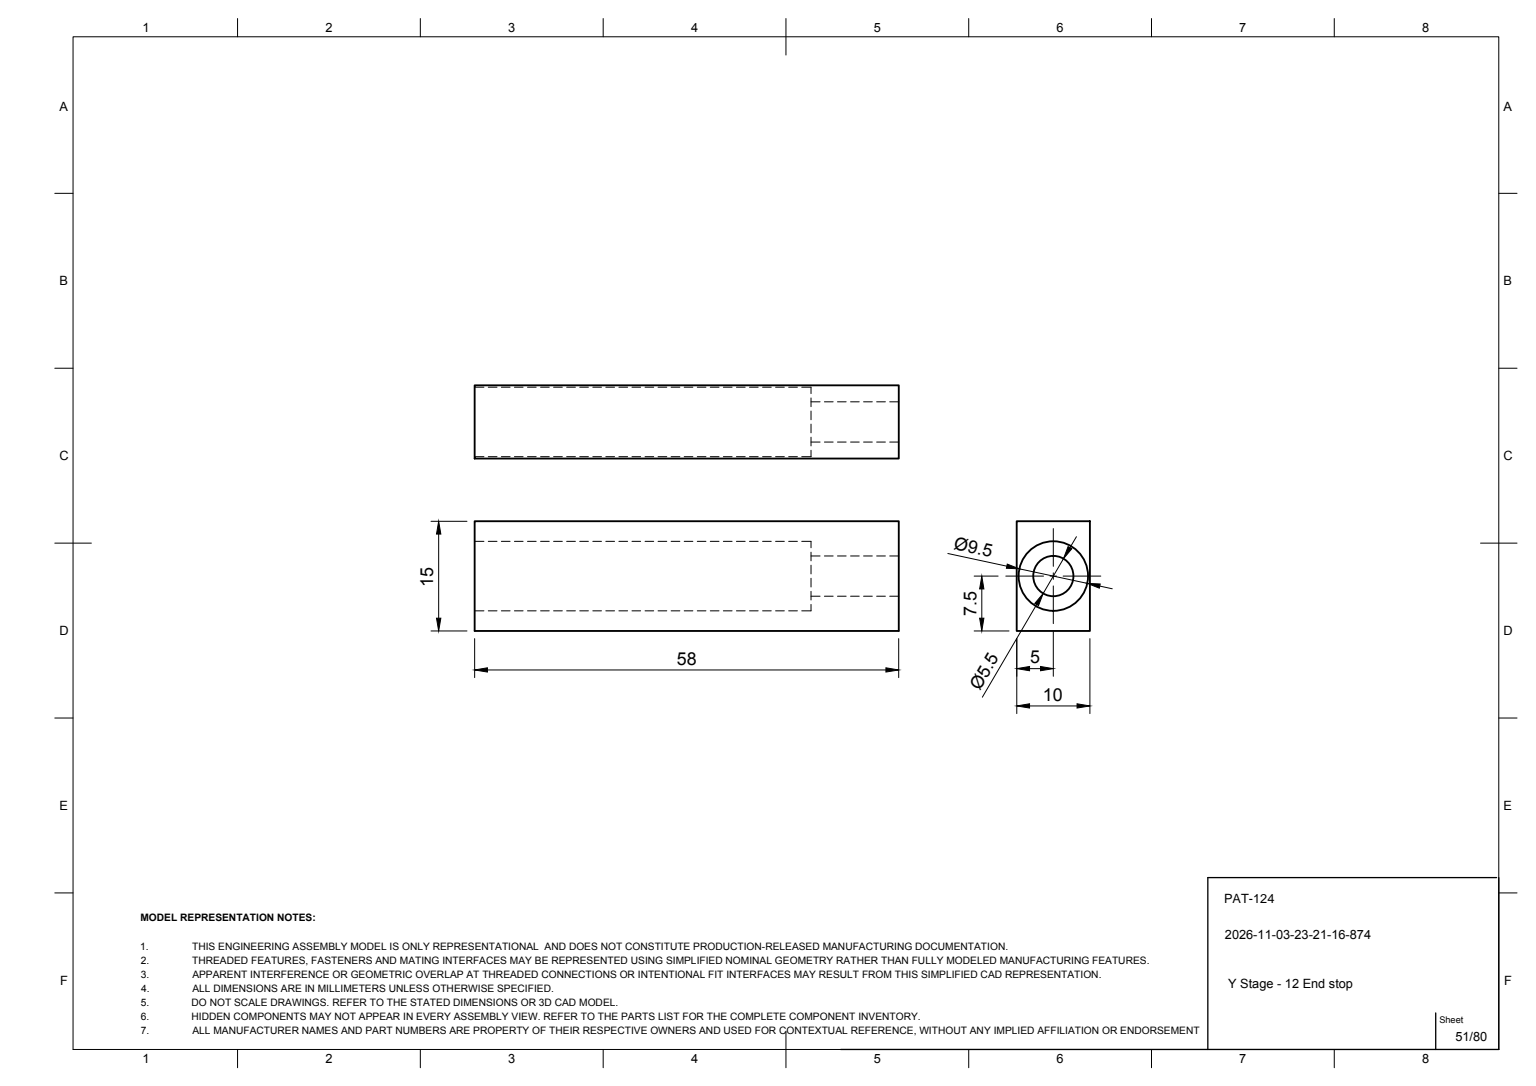
ISO-10303-21;
HEADER;
/* Generated by software containing ST-Developer
 * from STEP Tools, Inc. (www.steptools.com) 
 */

FILE_DESCRIPTION(
/* description */ ('XY cross-slide table'),
/* implementation_level */ '2;1');

FILE_NAME(
/* name */ 'Y Stage - 12 End stop.step',
/* time_stamp */ '2026-10-28T03:22:46-07:00',
/* author */ (''),
/* organization */ (''),
/* preprocessor_version */ 'ST-DEVELOPER v20.2',
/* originating_system */ 'Autodesk Translation Framework v15.17.0.0',
/* authorisation */ '');

FILE_SCHEMA (('AUTOMOTIVE_DESIGN { 1 0 10303 214 3 1 1 }'));
ENDSEC;

DATA;
#10=MECHANICAL_DESIGN_GEOMETRIC_PRESENTATION_REPRESENTATION('',(#1733),#62984);
#1552=SHAPE_REPRESENTATION_RELATIONSHIP('SRR','None',#63407,#1635);
#1635=ADVANCED_BREP_SHAPE_REPRESENTATION('',(#1842),#62944);
#1733=STYLED_ITEM('',(#63905),#1842);
#1842=MANIFOLD_SOLID_BREP('Body1',#23031);
#2183=FACE_BOUND('',#5243,.T.);
#2184=FACE_BOUND('',#5250,.T.);
#2185=FACE_BOUND('',#5252,.T.);
#2630=PLANE('',#25463);
#2631=PLANE('',#25467);
#2632=PLANE('',#25468);
#2633=PLANE('',#25469);
#2634=PLANE('',#25470);
#2635=PLANE('',#25471);
#2636=PLANE('',#25472);
#3631=FACE_OUTER_BOUND('',#5241,.T.);
#3632=FACE_OUTER_BOUND('',#5242,.T.);
#3633=FACE_OUTER_BOUND('',#5244,.T.);
#3634=FACE_OUTER_BOUND('',#5245,.T.);
#3635=FACE_OUTER_BOUND('',#5246,.T.);
#3636=FACE_OUTER_BOUND('',#5247,.T.);
#3637=FACE_OUTER_BOUND('',#5248,.T.);
#3638=FACE_OUTER_BOUND('',#5249,.T.);
#3639=FACE_OUTER_BOUND('',#5251,.T.);
#5241=EDGE_LOOP('',(#18436,#18437,#18438,#18439));
#5242=EDGE_LOOP('',(#18440));
#5243=EDGE_LOOP('',(#18441));
#5244=EDGE_LOOP('',(#18442,#18443,#18444,#18445));
#5245=EDGE_LOOP('',(#18446,#18447,#18448,#18449));
#5246=EDGE_LOOP('',(#18450,#18451,#18452,#18453));
#5247=EDGE_LOOP('',(#18454,#18455,#18456,#18457));
#5248=EDGE_LOOP('',(#18458,#18459,#18460,#18461));
#5249=EDGE_LOOP('',(#18462,#18463,#18464,#18465));
#5250=EDGE_LOOP('',(#18466));
#5251=EDGE_LOOP('',(#18467,#18468,#18469,#18470));
#5252=EDGE_LOOP('',(#18471));
#6765=LINE('',#48330,#8252);
#6766=LINE('',#48338,#8253);
#6767=LINE('',#48342,#8254);
#6768=LINE('',#48344,#8255);
#6769=LINE('',#48346,#8256);
#6770=LINE('',#48347,#8257);
#6771=LINE('',#48350,#8258);
#6772=LINE('',#48352,#8259);
#6773=LINE('',#48353,#8260);
#6774=LINE('',#48356,#8261);
#6775=LINE('',#48358,#8262);
#6776=LINE('',#48359,#8263);
#6777=LINE('',#48361,#8264);
#6778=LINE('',#48362,#8265);
#8252=VECTOR('',#30244,0.475);
#8253=VECTOR('',#30255,0.275);
#8254=VECTOR('',#30258,1.);
#8255=VECTOR('',#30259,1.);
#8256=VECTOR('',#30260,1.);
#8257=VECTOR('',#30261,1.);
#8258=VECTOR('',#30264,1.);
#8259=VECTOR('',#30265,1.);
#8260=VECTOR('',#30266,1.);
#8261=VECTOR('',#30269,1.);
#8262=VECTOR('',#30270,1.);
#8263=VECTOR('',#30271,1.);
#8264=VECTOR('',#30274,1.);
#8265=VECTOR('',#30275,1.);
#9443=CIRCLE('',#25461,0.475);
#9444=CIRCLE('',#25462,0.475);
#9445=CIRCLE('',#25464,0.275);
#9446=CIRCLE('',#25466,0.275);
#10957=VERTEX_POINT('',#48327);
#10958=VERTEX_POINT('',#48329);
#10959=VERTEX_POINT('',#48333);
#10960=VERTEX_POINT('',#48336);
#10961=VERTEX_POINT('',#48340);
#10962=VERTEX_POINT('',#48341);
#10963=VERTEX_POINT('',#48343);
#10964=VERTEX_POINT('',#48345);
#10965=VERTEX_POINT('',#48349);
#10966=VERTEX_POINT('',#48351);
#10967=VERTEX_POINT('',#48355);
#10968=VERTEX_POINT('',#48357);
#13602=EDGE_CURVE('',#10957,#10957,#9443,.T.);
#13603=EDGE_CURVE('',#10957,#10958,#6765,.T.);
#13604=EDGE_CURVE('',#10958,#10958,#9444,.T.);
#13605=EDGE_CURVE('',#10959,#10959,#9445,.T.);
#13606=EDGE_CURVE('',#10960,#10960,#9446,.T.);
#13607=EDGE_CURVE('',#10960,#10959,#6766,.T.);
#13608=EDGE_CURVE('',#10961,#10962,#6767,.T.);
#13609=EDGE_CURVE('',#10962,#10963,#6768,.T.);
#13610=EDGE_CURVE('',#10964,#10963,#6769,.T.);
#13611=EDGE_CURVE('',#10961,#10964,#6770,.T.);
#13612=EDGE_CURVE('',#10965,#10961,#6771,.T.);
#13613=EDGE_CURVE('',#10966,#10964,#6772,.T.);
#13614=EDGE_CURVE('',#10965,#10966,#6773,.T.);
#13615=EDGE_CURVE('',#10967,#10965,#6774,.T.);
#13616=EDGE_CURVE('',#10968,#10966,#6775,.T.);
#13617=EDGE_CURVE('',#10967,#10968,#6776,.T.);
#13618=EDGE_CURVE('',#10962,#10967,#6777,.T.);
#13619=EDGE_CURVE('',#10963,#10968,#6778,.T.);
#18436=ORIENTED_EDGE('',*,*,#13602,.F.);
#18437=ORIENTED_EDGE('',*,*,#13603,.T.);
#18438=ORIENTED_EDGE('',*,*,#13604,.F.);
#18439=ORIENTED_EDGE('',*,*,#13603,.F.);
#18440=ORIENTED_EDGE('',*,*,#13602,.T.);
#18441=ORIENTED_EDGE('',*,*,#13605,.F.);
#18442=ORIENTED_EDGE('',*,*,#13606,.F.);
#18443=ORIENTED_EDGE('',*,*,#13607,.T.);
#18444=ORIENTED_EDGE('',*,*,#13605,.T.);
#18445=ORIENTED_EDGE('',*,*,#13607,.F.);
#18446=ORIENTED_EDGE('',*,*,#13608,.T.);
#18447=ORIENTED_EDGE('',*,*,#13609,.T.);
#18448=ORIENTED_EDGE('',*,*,#13610,.F.);
#18449=ORIENTED_EDGE('',*,*,#13611,.F.);
#18450=ORIENTED_EDGE('',*,*,#13612,.T.);
#18451=ORIENTED_EDGE('',*,*,#13611,.T.);
#18452=ORIENTED_EDGE('',*,*,#13613,.F.);
#18453=ORIENTED_EDGE('',*,*,#13614,.F.);
#18454=ORIENTED_EDGE('',*,*,#13615,.T.);
#18455=ORIENTED_EDGE('',*,*,#13614,.T.);
#18456=ORIENTED_EDGE('',*,*,#13616,.F.);
#18457=ORIENTED_EDGE('',*,*,#13617,.F.);
#18458=ORIENTED_EDGE('',*,*,#13618,.T.);
#18459=ORIENTED_EDGE('',*,*,#13617,.T.);
#18460=ORIENTED_EDGE('',*,*,#13619,.F.);
#18461=ORIENTED_EDGE('',*,*,#13609,.F.);
#18462=ORIENTED_EDGE('',*,*,#13619,.T.);
#18463=ORIENTED_EDGE('',*,*,#13616,.T.);
#18464=ORIENTED_EDGE('',*,*,#13613,.T.);
#18465=ORIENTED_EDGE('',*,*,#13610,.T.);
#18466=ORIENTED_EDGE('',*,*,#13604,.T.);
#18467=ORIENTED_EDGE('',*,*,#13618,.F.);
#18468=ORIENTED_EDGE('',*,*,#13608,.F.);
#18469=ORIENTED_EDGE('',*,*,#13612,.F.);
#18470=ORIENTED_EDGE('',*,*,#13615,.F.);
#18471=ORIENTED_EDGE('',*,*,#13606,.T.);
#21404=CYLINDRICAL_SURFACE('',#25460,0.475);
#21405=CYLINDRICAL_SURFACE('',#25465,0.275);
#22412=ADVANCED_FACE('',(#3631),#21404,.F.);
#22413=ADVANCED_FACE('',(#3632,#2183),#2630,.T.);
#22414=ADVANCED_FACE('',(#3633),#21405,.F.);
#22415=ADVANCED_FACE('',(#3634),#2631,.T.);
#22416=ADVANCED_FACE('',(#3635),#2632,.T.);
#22417=ADVANCED_FACE('',(#3636),#2633,.T.);
#22418=ADVANCED_FACE('',(#3637),#2634,.T.);
#22419=ADVANCED_FACE('',(#3638,#2184),#2635,.T.);
#22420=ADVANCED_FACE('',(#3639,#2185),#2636,.F.);
#23031=CLOSED_SHELL('',(#22412,#22413,#22414,#22415,#22416,#22417,#22418,
#22419,#22420));
#25459=AXIS2_PLACEMENT_3D('',#48325,#30238,#30239);
#25460=AXIS2_PLACEMENT_3D('',#48326,#30240,#30241);
#25461=AXIS2_PLACEMENT_3D('',#48328,#30242,#30243);
#25462=AXIS2_PLACEMENT_3D('',#48331,#30245,#30246);
#25463=AXIS2_PLACEMENT_3D('',#48332,#30247,#30248);
#25464=AXIS2_PLACEMENT_3D('',#48334,#30249,#30250);
#25465=AXIS2_PLACEMENT_3D('',#48335,#30251,#30252);
#25466=AXIS2_PLACEMENT_3D('',#48337,#30253,#30254);
#25467=AXIS2_PLACEMENT_3D('',#48339,#30256,#30257);
#25468=AXIS2_PLACEMENT_3D('',#48348,#30262,#30263);
#25469=AXIS2_PLACEMENT_3D('',#48354,#30267,#30268);
#25470=AXIS2_PLACEMENT_3D('',#48360,#30272,#30273);
#25471=AXIS2_PLACEMENT_3D('',#48363,#30276,#30277);
#25472=AXIS2_PLACEMENT_3D('',#48364,#30278,#30279);
#30238=DIRECTION('axis',(0.,0.,1.));
#30239=DIRECTION('refdir',(1.,0.,0.));
#30240=DIRECTION('center_axis',(0.,0.,1.));
#30241=DIRECTION('ref_axis',(1.,0.,0.));
#30242=DIRECTION('center_axis',(0.,0.,1.));
#30243=DIRECTION('ref_axis',(1.,0.,0.));
#30244=DIRECTION('',(0.,0.,1.));
#30245=DIRECTION('center_axis',(0.,0.,-1.));
#30246=DIRECTION('ref_axis',(1.,0.,0.));
#30247=DIRECTION('center_axis',(0.,0.,1.));
#30248=DIRECTION('ref_axis',(1.,0.,0.));
#30249=DIRECTION('center_axis',(0.,0.,1.));
#30250=DIRECTION('ref_axis',(1.,0.,0.));
#30251=DIRECTION('center_axis',(0.,0.,1.));
#30252=DIRECTION('ref_axis',(1.,0.,0.));
#30253=DIRECTION('center_axis',(0.,0.,1.));
#30254=DIRECTION('ref_axis',(1.,0.,0.));
#30255=DIRECTION('',(0.,0.,1.));
#30256=DIRECTION('center_axis',(0.,1.,0.));
#30257=DIRECTION('ref_axis',(-1.,0.,0.));
#30258=DIRECTION('',(-1.,0.,0.));
#30259=DIRECTION('',(0.,0.,1.));
#30260=DIRECTION('',(-1.,0.,0.));
#30261=DIRECTION('',(0.,0.,1.));
#30262=DIRECTION('center_axis',(1.,0.,0.));
#30263=DIRECTION('ref_axis',(0.,1.,0.));
#30264=DIRECTION('',(0.,1.,0.));
#30265=DIRECTION('',(0.,1.,0.));
#30266=DIRECTION('',(0.,0.,1.));
#30267=DIRECTION('center_axis',(0.,-1.,0.));
#30268=DIRECTION('ref_axis',(1.,0.,0.));
#30269=DIRECTION('',(1.,0.,0.));
#30270=DIRECTION('',(1.,0.,0.));
#30271=DIRECTION('',(0.,0.,1.));
#30272=DIRECTION('center_axis',(-1.,0.,0.));
#30273=DIRECTION('ref_axis',(0.,-1.,0.));
#30274=DIRECTION('',(0.,-1.,0.));
#30275=DIRECTION('',(0.,-1.,0.));
#30276=DIRECTION('center_axis',(0.,0.,1.));
#30277=DIRECTION('ref_axis',(1.,0.,0.));
#30278=DIRECTION('center_axis',(0.,0.,1.));
#30279=DIRECTION('ref_axis',(1.,0.,0.));
#48325=CARTESIAN_POINT('',(0.,0.,0.));
#48326=CARTESIAN_POINT('Origin',(3.5,-9.25,2.4));
#48327=CARTESIAN_POINT('',(3.025,-9.25,2.4));
#48328=CARTESIAN_POINT('Origin',(3.5,-9.25,2.4));
#48329=CARTESIAN_POINT('',(3.025,-9.25,7.));
#48330=CARTESIAN_POINT('',(3.025,-9.25,2.4));
#48331=CARTESIAN_POINT('Origin',(3.5,-9.25,7.));
#48332=CARTESIAN_POINT('Origin',(3.5,-9.25,2.4));
#48333=CARTESIAN_POINT('',(3.225,-9.25,2.4));
#48334=CARTESIAN_POINT('Origin',(3.5,-9.25,2.4));
#48335=CARTESIAN_POINT('Origin',(3.5,-9.25,1.1));
#48336=CARTESIAN_POINT('',(3.225,-9.25,1.2));
#48337=CARTESIAN_POINT('Origin',(3.5,-9.25,1.2));
#48338=CARTESIAN_POINT('',(3.225,-9.25,1.1));
#48339=CARTESIAN_POINT('Origin',(4.,-8.5,1.2));
#48340=CARTESIAN_POINT('',(4.,-8.5,1.2));
#48341=CARTESIAN_POINT('',(3.,-8.5,1.2));
#48342=CARTESIAN_POINT('',(4.,-8.5,1.2));
#48343=CARTESIAN_POINT('',(3.,-8.5,7.));
#48344=CARTESIAN_POINT('',(3.,-8.5,1.2));
#48345=CARTESIAN_POINT('',(4.,-8.5,7.));
#48346=CARTESIAN_POINT('',(4.,-8.5,7.));
#48347=CARTESIAN_POINT('',(4.,-8.5,1.2));
#48348=CARTESIAN_POINT('Origin',(4.,-10.,1.2));
#48349=CARTESIAN_POINT('',(4.,-10.,1.2));
#48350=CARTESIAN_POINT('',(4.,-10.,1.2));
#48351=CARTESIAN_POINT('',(4.,-10.,7.));
#48352=CARTESIAN_POINT('',(4.,-10.,7.));
#48353=CARTESIAN_POINT('',(4.,-10.,1.2));
#48354=CARTESIAN_POINT('Origin',(3.,-10.,1.2));
#48355=CARTESIAN_POINT('',(3.,-10.,1.2));
#48356=CARTESIAN_POINT('',(3.,-10.,1.2));
#48357=CARTESIAN_POINT('',(3.,-10.,7.));
#48358=CARTESIAN_POINT('',(3.,-10.,7.));
#48359=CARTESIAN_POINT('',(3.,-10.,1.2));
#48360=CARTESIAN_POINT('Origin',(3.,-8.5,1.2));
#48361=CARTESIAN_POINT('',(3.,-8.5,1.2));
#48362=CARTESIAN_POINT('',(3.,-8.5,7.));
#48363=CARTESIAN_POINT('Origin',(3.5,-9.25,7.));
#48364=CARTESIAN_POINT('Origin',(3.5,-9.25,1.2));
#62845=UNCERTAINTY_MEASURE_WITH_UNIT(LENGTH_MEASURE(0.001),#62985,
'DISTANCE_ACCURACY_VALUE',
'Maximum model space distance between geometric entities at asserted c
onnectivities');
#62885=UNCERTAINTY_MEASURE_WITH_UNIT(LENGTH_MEASURE(0.001),#62985,
'DISTANCE_ACCURACY_VALUE',
'Maximum model space distance between geometric entities at asserted c
onnectivities');
#62944=(
GEOMETRIC_REPRESENTATION_CONTEXT(3)
GLOBAL_UNCERTAINTY_ASSIGNED_CONTEXT((#62845))
GLOBAL_UNIT_ASSIGNED_CONTEXT((#62985,#62987,#62988))
REPRESENTATION_CONTEXT('','3D')
);
#62984=(
GEOMETRIC_REPRESENTATION_CONTEXT(3)
GLOBAL_UNCERTAINTY_ASSIGNED_CONTEXT((#62885))
GLOBAL_UNIT_ASSIGNED_CONTEXT((#62985,#62987,#62988))
REPRESENTATION_CONTEXT('','3D')
);
#62985=(
LENGTH_UNIT()
NAMED_UNIT(*)
SI_UNIT(.CENTI.,.METRE.)
);
#62987=(
NAMED_UNIT(*)
PLANE_ANGLE_UNIT()
SI_UNIT($,.RADIAN.)
);
#62988=(
NAMED_UNIT(*)
SI_UNIT($,.STERADIAN.)
SOLID_ANGLE_UNIT()
);
#63047=SHAPE_DEFINITION_REPRESENTATION(#63225,#63407);
#63225=PRODUCT_DEFINITION_SHAPE('',$,#63506);
#63407=SHAPE_REPRESENTATION('',(#25459),#62944);
#63447=PRODUCT_DEFINITION_CONTEXT('part definition',#63743,'design');
#63506=PRODUCT_DEFINITION('Y Stage - 12 End stop',
'Y Stage - 12 End stop',#63604,#63447);
#63604=PRODUCT_DEFINITION_FORMATION('',$,#63803);
#63743=APPLICATION_CONTEXT(
'Core Data for Automotive Mechanical Design Process');
#63744=PRODUCT_CONTEXT('part definition',#63743,'mechanical');
#63803=PRODUCT('Y Stage - 12 End stop','Y Stage - 12 End stop',
'Y Stage - 12 End stop',(#63744));
#63899=COLOUR_RGB('Sky Blue',0.24,0.69,0.87);
#63900=FILL_AREA_STYLE_COLOUR('',#63899);
#63901=FILL_AREA_STYLE('',(#63900));
#63902=SURFACE_STYLE_FILL_AREA(#63901);
#63903=SURFACE_SIDE_STYLE('',(#63902));
#63904=SURFACE_STYLE_USAGE(.BOTH.,#63903);
#63905=PRESENTATION_STYLE_ASSIGNMENT((#63904));
ENDSEC;
END-ISO-10303-21;
